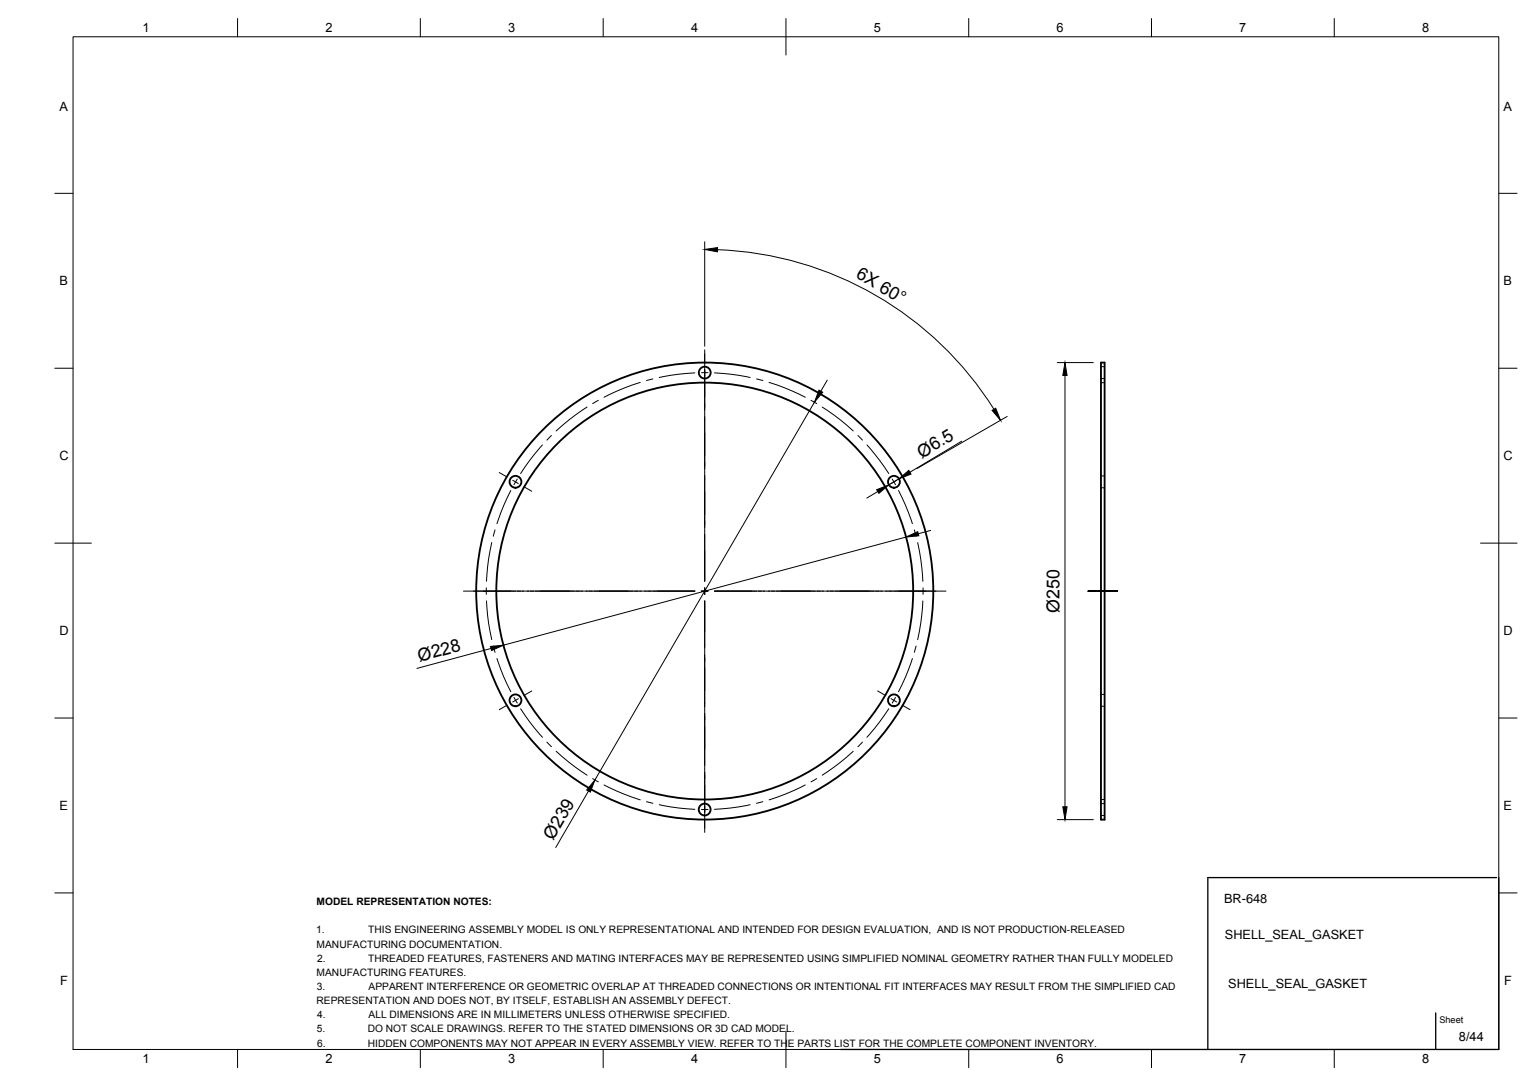
ISO-10303-21;
HEADER;
FILE_DESCRIPTION((''),'2;1');
FILE_NAME('SHELL_SEAL_GASKET.step','2026-10-01T22:05:39-07:00',(''),(''),'','','');
FILE_SCHEMA (('AUTOMOTIVE_DESIGN { 1 0 10303 214 3 1 1 }'));
ENDSEC;
DATA;
#10=MECHANICAL_DESIGN_GEOMETRIC_PRESENTATION_REPRESENTATION('',(#608),#24628);
#524=SHAPE_REPRESENTATION_RELATIONSHIP('SRR','None',#24796,#566) ;
#566=ADVANCED_BREP_SHAPE_REPRESENTATION('',(#650),#24586) ;
#608=STYLED_ITEM('',(#25033),#650) ;
#650=MANIFOLD_SOLID_BREP('SHELL_SEAL_GASKET',#13117) ;
#735=FACE_BOUND('',#3842,.T.) ;
#736=FACE_BOUND('',#3843,.T.) ;
#737=FACE_BOUND('',#3844,.T.) ;
#738=FACE_BOUND('',#3845,.T.) ;
#739=FACE_BOUND('',#3846,.T.) ;
#740=FACE_BOUND('',#3847,.T.) ;
#741=FACE_BOUND('',#3848,.T.) ;
#742=FACE_BOUND('',#3850,.T.) ;
#743=FACE_BOUND('',#3851,.T.) ;
#744=FACE_BOUND('',#3852,.T.) ;
#745=FACE_BOUND('',#3853,.T.) ;
#746=FACE_BOUND('',#3854,.T.) ;
#747=FACE_BOUND('',#3855,.T.) ;
#748=FACE_BOUND('',#3856,.T.) ;
#1063=LINE('',#20139,#1899) ;
#1064=LINE('',#20145,#1900) ;
#1065=LINE('',#20151,#1901) ;
#1066=LINE('',#20157,#1902) ;
#1067=LINE('',#20163,#1903) ;
#1068=LINE('',#20169,#1904) ;
#1069=LINE('',#20175,#1905) ;
#1070=LINE('',#20181,#1906) ;
#1899=VECTOR('',#15776,0.325) ;
#1900=VECTOR('',#15783,0.325) ;
#1901=VECTOR('',#15790,0.325) ;
#1902=VECTOR('',#15797,0.325) ;
#1903=VECTOR('',#15804,0.325) ;
#1904=VECTOR('',#15811,0.325) ;
#1905=VECTOR('',#15818,11.4) ;
#1906=VECTOR('',#15825,12.5) ;
#2709=CYLINDRICAL_SURFACE('',#13812,0.325) ;
#2710=CYLINDRICAL_SURFACE('',#13815,0.325) ;
#2711=CYLINDRICAL_SURFACE('',#13818,0.325) ;
#2712=CYLINDRICAL_SURFACE('',#13821,0.325) ;
#2713=CYLINDRICAL_SURFACE('',#13824,0.325) ;
#2714=CYLINDRICAL_SURFACE('',#13827,0.325) ;
#2715=CYLINDRICAL_SURFACE('',#13830,11.4) ;
#2716=CYLINDRICAL_SURFACE('',#13833,12.5) ;
#3017=FACE_OUTER_BOUND('',#3833,.T.) ;
#3018=FACE_OUTER_BOUND('',#3834,.T.) ;
#3019=FACE_OUTER_BOUND('',#3835,.T.) ;
#3020=FACE_OUTER_BOUND('',#3836,.T.) ;
#3021=FACE_OUTER_BOUND('',#3837,.T.) ;
#3022=FACE_OUTER_BOUND('',#3838,.T.) ;
#3023=FACE_OUTER_BOUND('',#3839,.T.) ;
#3024=FACE_OUTER_BOUND('',#3840,.T.) ;
#3025=FACE_OUTER_BOUND('',#3841,.T.) ;
#3026=FACE_OUTER_BOUND('',#3849,.T.) ;
#3833=EDGE_LOOP('',(#8799,#8800,#8801,#8802)) ;
#3834=EDGE_LOOP('',(#8803,#8804,#8805,#8806)) ;
#3835=EDGE_LOOP('',(#8807,#8808,#8809,#8810)) ;
#3836=EDGE_LOOP('',(#8811,#8812,#8813,#8814)) ;
#3837=EDGE_LOOP('',(#8815,#8816,#8817,#8818)) ;
#3838=EDGE_LOOP('',(#8819,#8820,#8821,#8822)) ;
#3839=EDGE_LOOP('',(#8823,#8824,#8825,#8826)) ;
#3840=EDGE_LOOP('',(#8827,#8828,#8829,#8830)) ;
#3841=EDGE_LOOP('',(#8831)) ;
#3842=EDGE_LOOP('',(#8832)) ;
#3843=EDGE_LOOP('',(#8833)) ;
#3844=EDGE_LOOP('',(#8834)) ;
#3845=EDGE_LOOP('',(#8835)) ;
#3846=EDGE_LOOP('',(#8836)) ;
#3847=EDGE_LOOP('',(#8837)) ;
#3848=EDGE_LOOP('',(#8838)) ;
#3849=EDGE_LOOP('',(#8839)) ;
#3850=EDGE_LOOP('',(#8840)) ;
#3851=EDGE_LOOP('',(#8841)) ;
#3852=EDGE_LOOP('',(#8842)) ;
#3853=EDGE_LOOP('',(#8843)) ;
#3854=EDGE_LOOP('',(#8844)) ;
#3855=EDGE_LOOP('',(#8845)) ;
#3856=EDGE_LOOP('',(#8846)) ;
#4840=CIRCLE('',#13813,0.325) ;
#4841=CIRCLE('',#13814,0.325) ;
#4842=CIRCLE('',#13816,0.325) ;
#4843=CIRCLE('',#13817,0.325) ;
#4844=CIRCLE('',#13819,0.325) ;
#4845=CIRCLE('',#13820,0.325) ;
#4846=CIRCLE('',#13822,0.325) ;
#4847=CIRCLE('',#13823,0.325) ;
#4848=CIRCLE('',#13825,0.325) ;
#4849=CIRCLE('',#13826,0.325) ;
#4850=CIRCLE('',#13828,0.325) ;
#4851=CIRCLE('',#13829,0.325) ;
#4852=CIRCLE('',#13831,11.4) ;
#4853=CIRCLE('',#13832,11.4) ;
#4854=CIRCLE('',#13834,12.5) ;
#4855=CIRCLE('',#13835,12.5) ;
#5641=VERTEX_POINT('',#20136) ;
#5642=VERTEX_POINT('',#20138) ;
#5643=VERTEX_POINT('',#20142) ;
#5644=VERTEX_POINT('',#20144) ;
#5645=VERTEX_POINT('',#20148) ;
#5646=VERTEX_POINT('',#20150) ;
#5647=VERTEX_POINT('',#20154) ;
#5648=VERTEX_POINT('',#20156) ;
#5649=VERTEX_POINT('',#20160) ;
#5650=VERTEX_POINT('',#20162) ;
#5651=VERTEX_POINT('',#20166) ;
#5652=VERTEX_POINT('',#20168) ;
#5653=VERTEX_POINT('',#20172) ;
#5654=VERTEX_POINT('',#20174) ;
#5655=VERTEX_POINT('',#20178) ;
#5656=VERTEX_POINT('',#20180) ;
#6889=EDGE_CURVE('',#5641,#5641,#4840,.T.) ;
#6890=EDGE_CURVE('',#5641,#5642,#1063,.T.) ;
#6891=EDGE_CURVE('',#5642,#5642,#4841,.T.) ;
#6892=EDGE_CURVE('',#5643,#5643,#4842,.T.) ;
#6893=EDGE_CURVE('',#5643,#5644,#1064,.T.) ;
#6894=EDGE_CURVE('',#5644,#5644,#4843,.T.) ;
#6895=EDGE_CURVE('',#5645,#5645,#4844,.T.) ;
#6896=EDGE_CURVE('',#5645,#5646,#1065,.T.) ;
#6897=EDGE_CURVE('',#5646,#5646,#4845,.T.) ;
#6898=EDGE_CURVE('',#5647,#5647,#4846,.T.) ;
#6899=EDGE_CURVE('',#5647,#5648,#1066,.T.) ;
#6900=EDGE_CURVE('',#5648,#5648,#4847,.T.) ;
#6901=EDGE_CURVE('',#5649,#5649,#4848,.T.) ;
#6902=EDGE_CURVE('',#5649,#5650,#1067,.T.) ;
#6903=EDGE_CURVE('',#5650,#5650,#4849,.T.) ;
#6904=EDGE_CURVE('',#5651,#5651,#4850,.T.) ;
#6905=EDGE_CURVE('',#5651,#5652,#1068,.T.) ;
#6906=EDGE_CURVE('',#5652,#5652,#4851,.T.) ;
#6907=EDGE_CURVE('',#5653,#5653,#4852,.T.) ;
#6908=EDGE_CURVE('',#5653,#5654,#1069,.T.) ;
#6909=EDGE_CURVE('',#5654,#5654,#4853,.T.) ;
#6910=EDGE_CURVE('',#5655,#5655,#4854,.T.) ;
#6911=EDGE_CURVE('',#5655,#5656,#1070,.T.) ;
#6912=EDGE_CURVE('',#5656,#5656,#4855,.T.) ;
#8799=ORIENTED_EDGE('',*,*,#6889,.F.) ;
#8800=ORIENTED_EDGE('',*,*,#6890,.T.) ;
#8801=ORIENTED_EDGE('',*,*,#6891,.F.) ;
#8802=ORIENTED_EDGE('',*,*,#6890,.F.) ;
#8803=ORIENTED_EDGE('',*,*,#6892,.F.) ;
#8804=ORIENTED_EDGE('',*,*,#6893,.T.) ;
#8805=ORIENTED_EDGE('',*,*,#6894,.F.) ;
#8806=ORIENTED_EDGE('',*,*,#6893,.F.) ;
#8807=ORIENTED_EDGE('',*,*,#6895,.F.) ;
#8808=ORIENTED_EDGE('',*,*,#6896,.T.) ;
#8809=ORIENTED_EDGE('',*,*,#6897,.F.) ;
#8810=ORIENTED_EDGE('',*,*,#6896,.F.) ;
#8811=ORIENTED_EDGE('',*,*,#6898,.F.) ;
#8812=ORIENTED_EDGE('',*,*,#6899,.T.) ;
#8813=ORIENTED_EDGE('',*,*,#6900,.F.) ;
#8814=ORIENTED_EDGE('',*,*,#6899,.F.) ;
#8815=ORIENTED_EDGE('',*,*,#6901,.F.) ;
#8816=ORIENTED_EDGE('',*,*,#6902,.T.) ;
#8817=ORIENTED_EDGE('',*,*,#6903,.F.) ;
#8818=ORIENTED_EDGE('',*,*,#6902,.F.) ;
#8819=ORIENTED_EDGE('',*,*,#6904,.F.) ;
#8820=ORIENTED_EDGE('',*,*,#6905,.T.) ;
#8821=ORIENTED_EDGE('',*,*,#6906,.F.) ;
#8822=ORIENTED_EDGE('',*,*,#6905,.F.) ;
#8823=ORIENTED_EDGE('',*,*,#6907,.F.) ;
#8824=ORIENTED_EDGE('',*,*,#6908,.T.) ;
#8825=ORIENTED_EDGE('',*,*,#6909,.F.) ;
#8826=ORIENTED_EDGE('',*,*,#6908,.F.) ;
#8827=ORIENTED_EDGE('',*,*,#6910,.F.) ;
#8828=ORIENTED_EDGE('',*,*,#6911,.T.) ;
#8829=ORIENTED_EDGE('',*,*,#6912,.F.) ;
#8830=ORIENTED_EDGE('',*,*,#6911,.F.) ;
#8831=ORIENTED_EDGE('',*,*,#6912,.T.) ;
#8832=ORIENTED_EDGE('',*,*,#6889,.T.) ;
#8833=ORIENTED_EDGE('',*,*,#6892,.T.) ;
#8834=ORIENTED_EDGE('',*,*,#6895,.T.) ;
#8835=ORIENTED_EDGE('',*,*,#6898,.T.) ;
#8836=ORIENTED_EDGE('',*,*,#6901,.T.) ;
#8837=ORIENTED_EDGE('',*,*,#6904,.T.) ;
#8838=ORIENTED_EDGE('',*,*,#6907,.T.) ;
#8839=ORIENTED_EDGE('',*,*,#6910,.T.) ;
#8840=ORIENTED_EDGE('',*,*,#6891,.T.) ;
#8841=ORIENTED_EDGE('',*,*,#6894,.T.) ;
#8842=ORIENTED_EDGE('',*,*,#6897,.T.) ;
#8843=ORIENTED_EDGE('',*,*,#6900,.T.) ;
#8844=ORIENTED_EDGE('',*,*,#6903,.T.) ;
#8845=ORIENTED_EDGE('',*,*,#6906,.T.) ;
#8846=ORIENTED_EDGE('',*,*,#6909,.T.) ;
#12024=PLANE('',#13836) ;
#12025=PLANE('',#13837) ;
#12412=ADVANCED_FACE('',(#3017),#2709,.F.) ;
#12413=ADVANCED_FACE('',(#3018),#2710,.F.) ;
#12414=ADVANCED_FACE('',(#3019),#2711,.F.) ;
#12415=ADVANCED_FACE('',(#3020),#2712,.F.) ;
#12416=ADVANCED_FACE('',(#3021),#2713,.F.) ;
#12417=ADVANCED_FACE('',(#3022),#2714,.F.) ;
#12418=ADVANCED_FACE('',(#3023),#2715,.F.) ;
#12419=ADVANCED_FACE('',(#3024),#2716,.T.) ;
#12420=ADVANCED_FACE('',(#3025,#735,#736,#737,#738,#739,#740,#741),#12024,
 .T.) ;
#12421=ADVANCED_FACE('',(#3026,#742,#743,#744,#745,#746,#747,#748),#12025,
 .T.) ;
#13117=CLOSED_SHELL('',(#12412,#12413,#12414,#12415,#12416,#12417,#12418,
#12419,#12420,#12421)) ;
#13811=AXIS2_PLACEMENT_3D('',#20134,#15770,#15771) ;
#13812=AXIS2_PLACEMENT_3D('',#20135,#15772,#15773) ;
#13813=AXIS2_PLACEMENT_3D('',#20137,#15774,#15775) ;
#13814=AXIS2_PLACEMENT_3D('',#20140,#15777,#15778) ;
#13815=AXIS2_PLACEMENT_3D('',#20141,#15779,#15780) ;
#13816=AXIS2_PLACEMENT_3D('',#20143,#15781,#15782) ;
#13817=AXIS2_PLACEMENT_3D('',#20146,#15784,#15785) ;
#13818=AXIS2_PLACEMENT_3D('',#20147,#15786,#15787) ;
#13819=AXIS2_PLACEMENT_3D('',#20149,#15788,#15789) ;
#13820=AXIS2_PLACEMENT_3D('',#20152,#15791,#15792) ;
#13821=AXIS2_PLACEMENT_3D('',#20153,#15793,#15794) ;
#13822=AXIS2_PLACEMENT_3D('',#20155,#15795,#15796) ;
#13823=AXIS2_PLACEMENT_3D('',#20158,#15798,#15799) ;
#13824=AXIS2_PLACEMENT_3D('',#20159,#15800,#15801) ;
#13825=AXIS2_PLACEMENT_3D('',#20161,#15802,#15803) ;
#13826=AXIS2_PLACEMENT_3D('',#20164,#15805,#15806) ;
#13827=AXIS2_PLACEMENT_3D('',#20165,#15807,#15808) ;
#13828=AXIS2_PLACEMENT_3D('',#20167,#15809,#15810) ;
#13829=AXIS2_PLACEMENT_3D('',#20170,#15812,#15813) ;
#13830=AXIS2_PLACEMENT_3D('',#20171,#15814,#15815) ;
#13831=AXIS2_PLACEMENT_3D('',#20173,#15816,#15817) ;
#13832=AXIS2_PLACEMENT_3D('',#20176,#15819,#15820) ;
#13833=AXIS2_PLACEMENT_3D('',#20177,#15821,#15822) ;
#13834=AXIS2_PLACEMENT_3D('',#20179,#15823,#15824) ;
#13835=AXIS2_PLACEMENT_3D('',#20182,#15826,#15827) ;
#13836=AXIS2_PLACEMENT_3D('',#20183,#15828,#15829) ;
#13837=AXIS2_PLACEMENT_3D('',#20184,#15830,#15831) ;
#15770=DIRECTION('axis',(0.,0.,1.)) ;
#15771=DIRECTION('refdir',(1.,0.,0.)) ;
#15772=DIRECTION('center_axis',(0.,1.,0.)) ;
#15773=DIRECTION('ref_axis',(1.,0.,0.)) ;
#15774=DIRECTION('center_axis',(0.,1.,0.)) ;
#15775=DIRECTION('ref_axis',(1.,0.,0.)) ;
#15776=DIRECTION('',(0.,1.,0.)) ;
#15777=DIRECTION('center_axis',(0.,-1.,0.)) ;
#15778=DIRECTION('ref_axis',(1.,0.,0.)) ;
#15779=DIRECTION('center_axis',(0.,1.,0.)) ;
#15780=DIRECTION('ref_axis',(1.,0.,0.)) ;
#15781=DIRECTION('center_axis',(0.,1.,0.)) ;
#15782=DIRECTION('ref_axis',(1.,0.,0.)) ;
#15783=DIRECTION('',(0.,1.,0.)) ;
#15784=DIRECTION('center_axis',(0.,-1.,0.)) ;
#15785=DIRECTION('ref_axis',(1.,0.,0.)) ;
#15786=DIRECTION('center_axis',(0.,1.,0.)) ;
#15787=DIRECTION('ref_axis',(1.,0.,0.)) ;
#15788=DIRECTION('center_axis',(0.,1.,0.)) ;
#15789=DIRECTION('ref_axis',(1.,0.,0.)) ;
#15790=DIRECTION('',(0.,1.,0.)) ;
#15791=DIRECTION('center_axis',(0.,-1.,0.)) ;
#15792=DIRECTION('ref_axis',(1.,0.,0.)) ;
#15793=DIRECTION('center_axis',(0.,1.,0.)) ;
#15794=DIRECTION('ref_axis',(1.,0.,0.)) ;
#15795=DIRECTION('center_axis',(0.,1.,0.)) ;
#15796=DIRECTION('ref_axis',(1.,0.,0.)) ;
#15797=DIRECTION('',(0.,1.,0.)) ;
#15798=DIRECTION('center_axis',(0.,-1.,0.)) ;
#15799=DIRECTION('ref_axis',(1.,0.,0.)) ;
#15800=DIRECTION('center_axis',(0.,1.,0.)) ;
#15801=DIRECTION('ref_axis',(1.,0.,0.)) ;
#15802=DIRECTION('center_axis',(0.,1.,0.)) ;
#15803=DIRECTION('ref_axis',(1.,0.,0.)) ;
#15804=DIRECTION('',(0.,1.,0.)) ;
#15805=DIRECTION('center_axis',(0.,-1.,0.)) ;
#15806=DIRECTION('ref_axis',(1.,0.,0.)) ;
#15807=DIRECTION('center_axis',(0.,1.,0.)) ;
#15808=DIRECTION('ref_axis',(1.,0.,0.)) ;
#15809=DIRECTION('center_axis',(0.,1.,0.)) ;
#15810=DIRECTION('ref_axis',(1.,0.,0.)) ;
#15811=DIRECTION('',(0.,1.,0.)) ;
#15812=DIRECTION('center_axis',(0.,-1.,0.)) ;
#15813=DIRECTION('ref_axis',(1.,0.,0.)) ;
#15814=DIRECTION('center_axis',(0.,1.,0.)) ;
#15815=DIRECTION('ref_axis',(1.,0.,0.)) ;
#15816=DIRECTION('center_axis',(0.,1.,0.)) ;
#15817=DIRECTION('ref_axis',(1.,0.,0.)) ;
#15818=DIRECTION('',(0.,1.,0.)) ;
#15819=DIRECTION('center_axis',(0.,-1.,0.)) ;
#15820=DIRECTION('ref_axis',(1.,0.,0.)) ;
#15821=DIRECTION('center_axis',(0.,1.,0.)) ;
#15822=DIRECTION('ref_axis',(1.,0.,0.)) ;
#15823=DIRECTION('center_axis',(0.,1.,0.)) ;
#15824=DIRECTION('ref_axis',(1.,0.,0.)) ;
#15825=DIRECTION('',(0.,-1.,0.)) ;
#15826=DIRECTION('center_axis',(0.,-1.,0.)) ;
#15827=DIRECTION('ref_axis',(1.,0.,0.)) ;
#15828=DIRECTION('center_axis',(0.,-1.,0.)) ;
#15829=DIRECTION('ref_axis',(-1.,0.,0.)) ;
#15830=DIRECTION('center_axis',(0.,1.,0.)) ;
#15831=DIRECTION('ref_axis',(1.,0.,0.)) ;
#20134=CARTESIAN_POINT('',(0.,0.,0.)) ;
#20135=CARTESIAN_POINT('Origin',(5.975,0.,-10.349003575224)) ;
#20136=CARTESIAN_POINT('',(5.65,-0.1,-10.349003575224)) ;
#20137=CARTESIAN_POINT('Origin',(5.975,-0.1,-10.349003575224)) ;
#20138=CARTESIAN_POINT('',(5.65,0.1,-10.349003575224)) ;
#20139=CARTESIAN_POINT('',(5.65,0.,-10.349003575224)) ;
#20140=CARTESIAN_POINT('Origin',(5.975,0.1,-10.349003575224)) ;
#20141=CARTESIAN_POINT('Origin',(-5.975,0.,-10.349003575224)) ;
#20142=CARTESIAN_POINT('',(-6.30000000000001,-0.1,-10.349003575224)) ;
#20143=CARTESIAN_POINT('Origin',(-5.975,-0.1,-10.349003575224)) ;
#20144=CARTESIAN_POINT('',(-6.30000000000001,0.1,-10.349003575224)) ;
#20145=CARTESIAN_POINT('',(-6.30000000000001,0.,-10.349003575224)) ;
#20146=CARTESIAN_POINT('Origin',(-5.975,0.1,-10.349003575224)) ;
#20147=CARTESIAN_POINT('Origin',(-11.95,0.,1.46345292498109E-15)) ;
#20148=CARTESIAN_POINT('',(-12.275,-0.1,1.50325394595338E-15)) ;
#20149=CARTESIAN_POINT('Origin',(-11.95,-0.1,1.46345292498109E-15)) ;
#20150=CARTESIAN_POINT('',(-12.275,0.1,1.4236519040088E-15)) ;
#20151=CARTESIAN_POINT('',(-12.275,0.,1.50325394595338E-15)) ;
#20152=CARTESIAN_POINT('Origin',(-11.95,0.1,1.46345292498109E-15)) ;
#20153=CARTESIAN_POINT('Origin',(-5.975,0.,10.349003575224)) ;
#20154=CARTESIAN_POINT('',(-6.3,-0.1,10.349003575224)) ;
#20155=CARTESIAN_POINT('Origin',(-5.975,-0.1,10.349003575224)) ;
#20156=CARTESIAN_POINT('',(-6.3,0.1,10.349003575224)) ;
#20157=CARTESIAN_POINT('',(-6.3,0.,10.349003575224)) ;
#20158=CARTESIAN_POINT('Origin',(-5.975,0.1,10.349003575224)) ;
#20159=CARTESIAN_POINT('Origin',(5.975,0.,10.349003575224)) ;
#20160=CARTESIAN_POINT('',(5.65,-0.1,10.349003575224)) ;
#20161=CARTESIAN_POINT('Origin',(5.975,-0.1,10.349003575224)) ;
#20162=CARTESIAN_POINT('',(5.65,0.1,10.349003575224)) ;
#20163=CARTESIAN_POINT('',(5.65,0.,10.349003575224)) ;
#20164=CARTESIAN_POINT('Origin',(5.975,0.1,10.349003575224)) ;
#20165=CARTESIAN_POINT('Origin',(11.95,0.,0.)) ;
#20166=CARTESIAN_POINT('',(11.625,-0.1,3.9801020972289E-17)) ;
#20167=CARTESIAN_POINT('Origin',(11.95,-0.1,0.)) ;
#20168=CARTESIAN_POINT('',(11.625,0.1,-3.9801020972289E-17)) ;
#20169=CARTESIAN_POINT('',(11.625,0.,3.9801020972289E-17)) ;
#20170=CARTESIAN_POINT('Origin',(11.95,0.1,0.)) ;
#20171=CARTESIAN_POINT('Origin',(0.,0.,0.)) ;
#20172=CARTESIAN_POINT('',(-11.4,-0.1,1.39609735102798E-15)) ;
#20173=CARTESIAN_POINT('Origin',(0.,-0.1,0.)) ;
#20174=CARTESIAN_POINT('',(-11.4,0.1,-1.39609735102798E-15)) ;
#20175=CARTESIAN_POINT('',(-11.4,0.,1.39609735102798E-15)) ;
#20176=CARTESIAN_POINT('Origin',(0.,0.1,0.)) ;
#20177=CARTESIAN_POINT('Origin',(0.,0.,0.)) ;
#20178=CARTESIAN_POINT('',(-12.5,0.1,1.53080849893419E-15)) ;
#20179=CARTESIAN_POINT('Origin',(0.,0.1,0.)) ;
#20180=CARTESIAN_POINT('',(-12.5,-0.1,1.53080849893419E-15)) ;
#20181=CARTESIAN_POINT('',(-12.5,0.,1.53080849893419E-15)) ;
#20182=CARTESIAN_POINT('Origin',(0.,-0.1,0.)) ;
#20183=CARTESIAN_POINT('Origin',(0.,-0.1,0.)) ;
#20184=CARTESIAN_POINT('Origin',(0.,0.1,0.)) ;
#24538=UNCERTAINTY_MEASURE_WITH_UNIT(LENGTH_MEASURE(0.001),#24629,
'DISTANCE_ACCURACY_VALUE',
'Maximum model space distance between geometric entities at asserted c
onnectivities') ;
#24580=UNCERTAINTY_MEASURE_WITH_UNIT(LENGTH_MEASURE(0.001),#24629,
'DISTANCE_ACCURACY_VALUE',
'Maximum model space distance between geometric entities at asserted c
onnectivities') ;
#24586=(
GEOMETRIC_REPRESENTATION_CONTEXT(3)
GLOBAL_UNCERTAINTY_ASSIGNED_CONTEXT((#24538))
GLOBAL_UNIT_ASSIGNED_CONTEXT((#24629,#24631,#24632))
REPRESENTATION_CONTEXT('','3D')
) ;
#24628=(
GEOMETRIC_REPRESENTATION_CONTEXT(3)
GLOBAL_UNCERTAINTY_ASSIGNED_CONTEXT((#24580))
GLOBAL_UNIT_ASSIGNED_CONTEXT((#24629,#24631,#24632))
REPRESENTATION_CONTEXT('','3D')
) ;
#24629=(
LENGTH_UNIT()
NAMED_UNIT(*)
SI_UNIT(.CENTI.,.METRE.)
) ;
#24631=(
NAMED_UNIT(*)
PLANE_ANGLE_UNIT()
SI_UNIT($,.RADIAN.)
) ;
#24632=(
NAMED_UNIT(*)
SI_UNIT($,.STERADIAN.)
SOLID_ANGLE_UNIT()
) ;
#24638=SHAPE_DEFINITION_REPRESENTATION(#24685,#24796) ;
#24685=PRODUCT_DEFINITION_SHAPE('',$,#24844) ;
#24796=SHAPE_REPRESENTATION('',(#13811),#24586) ;
#24838=PRODUCT_DEFINITION_CONTEXT('part definition',#24981,'design') ;
#24844=PRODUCT_DEFINITION('SHELL_SEAL_GASKET','SHELL_SEAL_GASKET',
#24891,#24838) ;
#24891=PRODUCT_DEFINITION_FORMATION('',$,#24988) ;
#24981=APPLICATION_CONTEXT(
'Core Data for Automotive Mechanical Design Process') ;
#24982=PRODUCT_CONTEXT('part definition',#24981,'mechanical') ;
#24988=PRODUCT('SHELL_SEAL_GASKET','SHELL_SEAL_GASKET',$,(#24982)) ;
#25033=PRESENTATION_STYLE_ASSIGNMENT((#25043)) ;
#25043=SURFACE_STYLE_USAGE(.BOTH.,#25053) ;
#25053=SURFACE_SIDE_STYLE('',(#25063)) ;
#25063=SURFACE_STYLE_FILL_AREA(#25073) ;
#25073=FILL_AREA_STYLE('Rubber - Soft',(#25083)) ;
#25083=FILL_AREA_STYLE_COLOUR('Rubber - Soft',#25093) ;
#25093=COLOUR_RGB('Rubber - Soft', 0.09019608, 0.27058824, 0.51372549) ;
ENDSEC;
END-ISO-10303-21;
